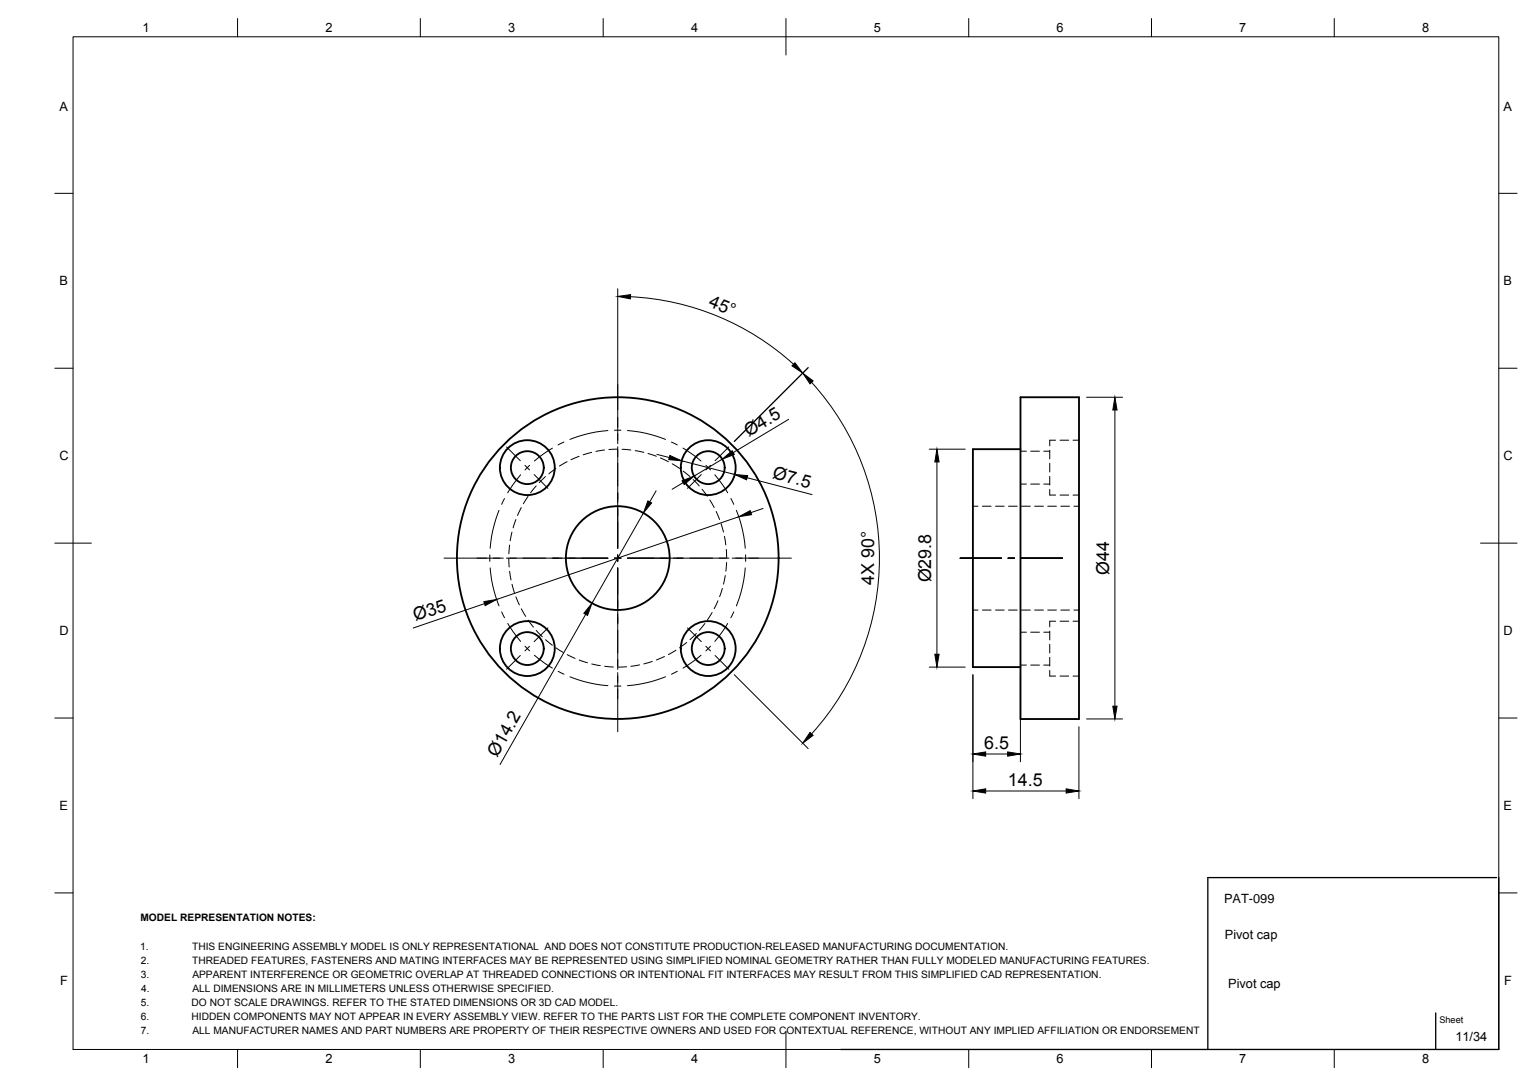
ISO-10303-21;
HEADER;
/* Generated by software containing ST-Developer
 * from STEP Tools, Inc. (www.steptools.com) 
 */

FILE_DESCRIPTION(
/* description */ ('PAT-099'),
/* implementation_level */ '2;1');

FILE_NAME(
/* name */ 'Pivot cap.step',
/* time_stamp */ '2026-10-29T17:25:42-07:00',
/* author */ (''),
/* organization */ (''),
/* preprocessor_version */ 'ST-DEVELOPER v20.2',
/* originating_system */ 'Autodesk Translation Framework v15.17.0.0',
/* authorisation */ '');

FILE_SCHEMA (('AUTOMOTIVE_DESIGN { 1 0 10303 214 3 1 1 }'));
ENDSEC;

DATA;
#10=MECHANICAL_DESIGN_GEOMETRIC_PRESENTATION_REPRESENTATION('',(#343),#11035);
#293=SHAPE_REPRESENTATION_RELATIONSHIP('SRR','None',#11161,#318);
#318=ADVANCED_BREP_SHAPE_REPRESENTATION('',(#376),#11011);
#343=STYLED_ITEM('',(#11372),#376);
#376=MANIFOLD_SOLID_BREP('Body1',#4711);
#463=FACE_BOUND('',#1091,.T.);
#464=FACE_BOUND('',#1094,.T.);
#465=FACE_BOUND('',#1097,.T.);
#466=FACE_BOUND('',#1100,.T.);
#467=FACE_BOUND('',#1107,.T.);
#468=FACE_BOUND('',#1111,.T.);
#469=FACE_BOUND('',#1112,.T.);
#470=FACE_BOUND('',#1113,.T.);
#471=FACE_BOUND('',#1114,.T.);
#472=FACE_BOUND('',#1115,.T.);
#473=FACE_BOUND('',#1117,.T.);
#474=FACE_BOUND('',#1118,.T.);
#475=FACE_BOUND('',#1119,.T.);
#476=FACE_BOUND('',#1120,.T.);
#477=FACE_BOUND('',#1121,.T.);
#555=PLANE('',#5222);
#556=PLANE('',#5227);
#557=PLANE('',#5232);
#558=PLANE('',#5237);
#559=PLANE('',#5250);
#560=PLANE('',#5257);
#561=PLANE('',#5258);
#746=FACE_OUTER_BOUND('',#1089,.T.);
#747=FACE_OUTER_BOUND('',#1090,.T.);
#748=FACE_OUTER_BOUND('',#1092,.T.);
#749=FACE_OUTER_BOUND('',#1093,.T.);
#750=FACE_OUTER_BOUND('',#1095,.T.);
#751=FACE_OUTER_BOUND('',#1096,.T.);
#752=FACE_OUTER_BOUND('',#1098,.T.);
#753=FACE_OUTER_BOUND('',#1099,.T.);
#754=FACE_OUTER_BOUND('',#1101,.T.);
#755=FACE_OUTER_BOUND('',#1102,.T.);
#756=FACE_OUTER_BOUND('',#1103,.T.);
#757=FACE_OUTER_BOUND('',#1104,.T.);
#758=FACE_OUTER_BOUND('',#1105,.T.);
#759=FACE_OUTER_BOUND('',#1106,.T.);
#760=FACE_OUTER_BOUND('',#1108,.T.);
#761=FACE_OUTER_BOUND('',#1109,.T.);
#762=FACE_OUTER_BOUND('',#1110,.T.);
#763=FACE_OUTER_BOUND('',#1116,.T.);
#1089=EDGE_LOOP('',(#3557,#3558,#3559,#3560));
#1090=EDGE_LOOP('',(#3561));
#1091=EDGE_LOOP('',(#3562));
#1092=EDGE_LOOP('',(#3563,#3564,#3565,#3566));
#1093=EDGE_LOOP('',(#3567));
#1094=EDGE_LOOP('',(#3568));
#1095=EDGE_LOOP('',(#3569,#3570,#3571,#3572));
#1096=EDGE_LOOP('',(#3573));
#1097=EDGE_LOOP('',(#3574));
#1098=EDGE_LOOP('',(#3575,#3576,#3577,#3578));
#1099=EDGE_LOOP('',(#3579));
#1100=EDGE_LOOP('',(#3580));
#1101=EDGE_LOOP('',(#3581,#3582,#3583,#3584));
#1102=EDGE_LOOP('',(#3585,#3586,#3587,#3588));
#1103=EDGE_LOOP('',(#3589,#3590,#3591,#3592));
#1104=EDGE_LOOP('',(#3593,#3594,#3595,#3596));
#1105=EDGE_LOOP('',(#3597,#3598,#3599,#3600));
#1106=EDGE_LOOP('',(#3601));
#1107=EDGE_LOOP('',(#3602));
#1108=EDGE_LOOP('',(#3603,#3604,#3605,#3606));
#1109=EDGE_LOOP('',(#3607,#3608,#3609,#3610));
#1110=EDGE_LOOP('',(#3611));
#1111=EDGE_LOOP('',(#3612));
#1112=EDGE_LOOP('',(#3613));
#1113=EDGE_LOOP('',(#3614));
#1114=EDGE_LOOP('',(#3615));
#1115=EDGE_LOOP('',(#3616));
#1116=EDGE_LOOP('',(#3617));
#1117=EDGE_LOOP('',(#3618));
#1118=EDGE_LOOP('',(#3619));
#1119=EDGE_LOOP('',(#3620));
#1120=EDGE_LOOP('',(#3621));
#1121=EDGE_LOOP('',(#3622));
#1425=LINE('',#9675,#1677);
#1426=LINE('',#9684,#1678);
#1427=LINE('',#9693,#1679);
#1428=LINE('',#9702,#1680);
#1429=LINE('',#9710,#1681);
#1430=LINE('',#9714,#1682);
#1431=LINE('',#9718,#1683);
#1432=LINE('',#9722,#1684);
#1433=LINE('',#9727,#1685);
#1434=LINE('',#9735,#1686);
#1435=LINE('',#9740,#1687);
#1677=VECTOR('',#6160,0.375);
#1678=VECTOR('',#6171,0.375);
#1679=VECTOR('',#6182,0.375);
#1680=VECTOR('',#6193,0.375);
#1681=VECTOR('',#6204,0.225);
#1682=VECTOR('',#6209,0.225);
#1683=VECTOR('',#6214,0.225);
#1684=VECTOR('',#6219,0.225);
#1685=VECTOR('',#6224,1.49);
#1686=VECTOR('',#6235,0.71);
#1687=VECTOR('',#6240,2.2);
#1955=CIRCLE('',#5220,0.375);
#1956=CIRCLE('',#5221,0.375);
#1957=CIRCLE('',#5223,0.225);
#1958=CIRCLE('',#5225,0.375);
#1959=CIRCLE('',#5226,0.375);
#1960=CIRCLE('',#5228,0.225);
#1961=CIRCLE('',#5230,0.375);
#1962=CIRCLE('',#5231,0.375);
#1963=CIRCLE('',#5233,0.225);
#1964=CIRCLE('',#5235,0.375);
#1965=CIRCLE('',#5236,0.375);
#1966=CIRCLE('',#5238,0.225);
#1967=CIRCLE('',#5240,0.225);
#1968=CIRCLE('',#5242,0.225);
#1969=CIRCLE('',#5244,0.225);
#1970=CIRCLE('',#5246,0.225);
#1971=CIRCLE('',#5248,1.49);
#1972=CIRCLE('',#5249,1.49);
#1973=CIRCLE('',#5251,0.71);
#1974=CIRCLE('',#5253,0.71);
#1975=CIRCLE('',#5255,2.2);
#1976=CIRCLE('',#5256,2.2);
#2284=VERTEX_POINT('',#9672);
#2285=VERTEX_POINT('',#9674);
#2286=VERTEX_POINT('',#9678);
#2287=VERTEX_POINT('',#9681);
#2288=VERTEX_POINT('',#9683);
#2289=VERTEX_POINT('',#9687);
#2290=VERTEX_POINT('',#9690);
#2291=VERTEX_POINT('',#9692);
#2292=VERTEX_POINT('',#9696);
#2293=VERTEX_POINT('',#9699);
#2294=VERTEX_POINT('',#9701);
#2295=VERTEX_POINT('',#9705);
#2296=VERTEX_POINT('',#9708);
#2297=VERTEX_POINT('',#9712);
#2298=VERTEX_POINT('',#9716);
#2299=VERTEX_POINT('',#9720);
#2300=VERTEX_POINT('',#9724);
#2301=VERTEX_POINT('',#9726);
#2302=VERTEX_POINT('',#9730);
#2303=VERTEX_POINT('',#9733);
#2304=VERTEX_POINT('',#9737);
#2305=VERTEX_POINT('',#9739);
#2755=EDGE_CURVE('',#2284,#2284,#1955,.T.);
#2756=EDGE_CURVE('',#2284,#2285,#1425,.T.);
#2757=EDGE_CURVE('',#2285,#2285,#1956,.T.);
#2758=EDGE_CURVE('',#2286,#2286,#1957,.T.);
#2759=EDGE_CURVE('',#2287,#2287,#1958,.T.);
#2760=EDGE_CURVE('',#2287,#2288,#1426,.T.);
#2761=EDGE_CURVE('',#2288,#2288,#1959,.T.);
#2762=EDGE_CURVE('',#2289,#2289,#1960,.T.);
#2763=EDGE_CURVE('',#2290,#2290,#1961,.T.);
#2764=EDGE_CURVE('',#2290,#2291,#1427,.T.);
#2765=EDGE_CURVE('',#2291,#2291,#1962,.T.);
#2766=EDGE_CURVE('',#2292,#2292,#1963,.T.);
#2767=EDGE_CURVE('',#2293,#2293,#1964,.T.);
#2768=EDGE_CURVE('',#2293,#2294,#1428,.T.);
#2769=EDGE_CURVE('',#2294,#2294,#1965,.T.);
#2770=EDGE_CURVE('',#2295,#2295,#1966,.T.);
#2771=EDGE_CURVE('',#2296,#2296,#1967,.T.);
#2772=EDGE_CURVE('',#2296,#2286,#1429,.T.);
#2773=EDGE_CURVE('',#2297,#2297,#1968,.T.);
#2774=EDGE_CURVE('',#2297,#2289,#1430,.T.);
#2775=EDGE_CURVE('',#2298,#2298,#1969,.T.);
#2776=EDGE_CURVE('',#2298,#2292,#1431,.T.);
#2777=EDGE_CURVE('',#2299,#2299,#1970,.T.);
#2778=EDGE_CURVE('',#2299,#2295,#1432,.T.);
#2779=EDGE_CURVE('',#2300,#2300,#1971,.T.);
#2780=EDGE_CURVE('',#2300,#2301,#1433,.T.);
#2781=EDGE_CURVE('',#2301,#2301,#1972,.T.);
#2782=EDGE_CURVE('',#2302,#2302,#1973,.T.);
#2783=EDGE_CURVE('',#2303,#2303,#1974,.T.);
#2784=EDGE_CURVE('',#2303,#2302,#1434,.T.);
#2785=EDGE_CURVE('',#2304,#2304,#1975,.T.);
#2786=EDGE_CURVE('',#2304,#2305,#1435,.T.);
#2787=EDGE_CURVE('',#2305,#2305,#1976,.T.);
#3557=ORIENTED_EDGE('',*,*,#2755,.F.);
#3558=ORIENTED_EDGE('',*,*,#2756,.T.);
#3559=ORIENTED_EDGE('',*,*,#2757,.F.);
#3560=ORIENTED_EDGE('',*,*,#2756,.F.);
#3561=ORIENTED_EDGE('',*,*,#2755,.T.);
#3562=ORIENTED_EDGE('',*,*,#2758,.F.);
#3563=ORIENTED_EDGE('',*,*,#2759,.F.);
#3564=ORIENTED_EDGE('',*,*,#2760,.T.);
#3565=ORIENTED_EDGE('',*,*,#2761,.F.);
#3566=ORIENTED_EDGE('',*,*,#2760,.F.);
#3567=ORIENTED_EDGE('',*,*,#2759,.T.);
#3568=ORIENTED_EDGE('',*,*,#2762,.F.);
#3569=ORIENTED_EDGE('',*,*,#2763,.F.);
#3570=ORIENTED_EDGE('',*,*,#2764,.T.);
#3571=ORIENTED_EDGE('',*,*,#2765,.F.);
#3572=ORIENTED_EDGE('',*,*,#2764,.F.);
#3573=ORIENTED_EDGE('',*,*,#2763,.T.);
#3574=ORIENTED_EDGE('',*,*,#2766,.F.);
#3575=ORIENTED_EDGE('',*,*,#2767,.F.);
#3576=ORIENTED_EDGE('',*,*,#2768,.T.);
#3577=ORIENTED_EDGE('',*,*,#2769,.F.);
#3578=ORIENTED_EDGE('',*,*,#2768,.F.);
#3579=ORIENTED_EDGE('',*,*,#2767,.T.);
#3580=ORIENTED_EDGE('',*,*,#2770,.F.);
#3581=ORIENTED_EDGE('',*,*,#2771,.F.);
#3582=ORIENTED_EDGE('',*,*,#2772,.T.);
#3583=ORIENTED_EDGE('',*,*,#2758,.T.);
#3584=ORIENTED_EDGE('',*,*,#2772,.F.);
#3585=ORIENTED_EDGE('',*,*,#2773,.F.);
#3586=ORIENTED_EDGE('',*,*,#2774,.T.);
#3587=ORIENTED_EDGE('',*,*,#2762,.T.);
#3588=ORIENTED_EDGE('',*,*,#2774,.F.);
#3589=ORIENTED_EDGE('',*,*,#2775,.F.);
#3590=ORIENTED_EDGE('',*,*,#2776,.T.);
#3591=ORIENTED_EDGE('',*,*,#2766,.T.);
#3592=ORIENTED_EDGE('',*,*,#2776,.F.);
#3593=ORIENTED_EDGE('',*,*,#2777,.F.);
#3594=ORIENTED_EDGE('',*,*,#2778,.T.);
#3595=ORIENTED_EDGE('',*,*,#2770,.T.);
#3596=ORIENTED_EDGE('',*,*,#2778,.F.);
#3597=ORIENTED_EDGE('',*,*,#2779,.F.);
#3598=ORIENTED_EDGE('',*,*,#2780,.T.);
#3599=ORIENTED_EDGE('',*,*,#2781,.T.);
#3600=ORIENTED_EDGE('',*,*,#2780,.F.);
#3601=ORIENTED_EDGE('',*,*,#2781,.F.);
#3602=ORIENTED_EDGE('',*,*,#2782,.F.);
#3603=ORIENTED_EDGE('',*,*,#2783,.F.);
#3604=ORIENTED_EDGE('',*,*,#2784,.T.);
#3605=ORIENTED_EDGE('',*,*,#2782,.T.);
#3606=ORIENTED_EDGE('',*,*,#2784,.F.);
#3607=ORIENTED_EDGE('',*,*,#2785,.F.);
#3608=ORIENTED_EDGE('',*,*,#2786,.T.);
#3609=ORIENTED_EDGE('',*,*,#2787,.T.);
#3610=ORIENTED_EDGE('',*,*,#2786,.F.);
#3611=ORIENTED_EDGE('',*,*,#2785,.T.);
#3612=ORIENTED_EDGE('',*,*,#2783,.T.);
#3613=ORIENTED_EDGE('',*,*,#2769,.T.);
#3614=ORIENTED_EDGE('',*,*,#2765,.T.);
#3615=ORIENTED_EDGE('',*,*,#2761,.T.);
#3616=ORIENTED_EDGE('',*,*,#2757,.T.);
#3617=ORIENTED_EDGE('',*,*,#2787,.F.);
#3618=ORIENTED_EDGE('',*,*,#2779,.T.);
#3619=ORIENTED_EDGE('',*,*,#2777,.T.);
#3620=ORIENTED_EDGE('',*,*,#2775,.T.);
#3621=ORIENTED_EDGE('',*,*,#2773,.T.);
#3622=ORIENTED_EDGE('',*,*,#2771,.T.);
#4363=CYLINDRICAL_SURFACE('',#5219,0.375);
#4364=CYLINDRICAL_SURFACE('',#5224,0.375);
#4365=CYLINDRICAL_SURFACE('',#5229,0.375);
#4366=CYLINDRICAL_SURFACE('',#5234,0.375);
#4367=CYLINDRICAL_SURFACE('',#5239,0.225);
#4368=CYLINDRICAL_SURFACE('',#5241,0.225);
#4369=CYLINDRICAL_SURFACE('',#5243,0.225);
#4370=CYLINDRICAL_SURFACE('',#5245,0.225);
#4371=CYLINDRICAL_SURFACE('',#5247,1.49);
#4372=CYLINDRICAL_SURFACE('',#5252,0.71);
#4373=CYLINDRICAL_SURFACE('',#5254,2.2);
#4511=ADVANCED_FACE('',(#746),#4363,.F.);
#4512=ADVANCED_FACE('',(#747,#463),#555,.T.);
#4513=ADVANCED_FACE('',(#748),#4364,.F.);
#4514=ADVANCED_FACE('',(#749,#464),#556,.T.);
#4515=ADVANCED_FACE('',(#750),#4365,.F.);
#4516=ADVANCED_FACE('',(#751,#465),#557,.T.);
#4517=ADVANCED_FACE('',(#752),#4366,.F.);
#4518=ADVANCED_FACE('',(#753,#466),#558,.T.);
#4519=ADVANCED_FACE('',(#754),#4367,.F.);
#4520=ADVANCED_FACE('',(#755),#4368,.F.);
#4521=ADVANCED_FACE('',(#756),#4369,.F.);
#4522=ADVANCED_FACE('',(#757),#4370,.F.);
#4523=ADVANCED_FACE('',(#758),#4371,.T.);
#4524=ADVANCED_FACE('',(#759,#467),#559,.F.);
#4525=ADVANCED_FACE('',(#760),#4372,.F.);
#4526=ADVANCED_FACE('',(#761),#4373,.T.);
#4527=ADVANCED_FACE('',(#762,#468,#469,#470,#471,#472),#560,.T.);
#4528=ADVANCED_FACE('',(#763,#473,#474,#475,#476,#477),#561,.F.);
#4711=CLOSED_SHELL('',(#4511,#4512,#4513,#4514,#4515,#4516,#4517,#4518,
#4519,#4520,#4521,#4522,#4523,#4524,#4525,#4526,#4527,#4528));
#5218=AXIS2_PLACEMENT_3D('',#9670,#6154,#6155);
#5219=AXIS2_PLACEMENT_3D('',#9671,#6156,#6157);
#5220=AXIS2_PLACEMENT_3D('',#9673,#6158,#6159);
#5221=AXIS2_PLACEMENT_3D('',#9676,#6161,#6162);
#5222=AXIS2_PLACEMENT_3D('',#9677,#6163,#6164);
#5223=AXIS2_PLACEMENT_3D('',#9679,#6165,#6166);
#5224=AXIS2_PLACEMENT_3D('',#9680,#6167,#6168);
#5225=AXIS2_PLACEMENT_3D('',#9682,#6169,#6170);
#5226=AXIS2_PLACEMENT_3D('',#9685,#6172,#6173);
#5227=AXIS2_PLACEMENT_3D('',#9686,#6174,#6175);
#5228=AXIS2_PLACEMENT_3D('',#9688,#6176,#6177);
#5229=AXIS2_PLACEMENT_3D('',#9689,#6178,#6179);
#5230=AXIS2_PLACEMENT_3D('',#9691,#6180,#6181);
#5231=AXIS2_PLACEMENT_3D('',#9694,#6183,#6184);
#5232=AXIS2_PLACEMENT_3D('',#9695,#6185,#6186);
#5233=AXIS2_PLACEMENT_3D('',#9697,#6187,#6188);
#5234=AXIS2_PLACEMENT_3D('',#9698,#6189,#6190);
#5235=AXIS2_PLACEMENT_3D('',#9700,#6191,#6192);
#5236=AXIS2_PLACEMENT_3D('',#9703,#6194,#6195);
#5237=AXIS2_PLACEMENT_3D('',#9704,#6196,#6197);
#5238=AXIS2_PLACEMENT_3D('',#9706,#6198,#6199);
#5239=AXIS2_PLACEMENT_3D('',#9707,#6200,#6201);
#5240=AXIS2_PLACEMENT_3D('',#9709,#6202,#6203);
#5241=AXIS2_PLACEMENT_3D('',#9711,#6205,#6206);
#5242=AXIS2_PLACEMENT_3D('',#9713,#6207,#6208);
#5243=AXIS2_PLACEMENT_3D('',#9715,#6210,#6211);
#5244=AXIS2_PLACEMENT_3D('',#9717,#6212,#6213);
#5245=AXIS2_PLACEMENT_3D('',#9719,#6215,#6216);
#5246=AXIS2_PLACEMENT_3D('',#9721,#6217,#6218);
#5247=AXIS2_PLACEMENT_3D('',#9723,#6220,#6221);
#5248=AXIS2_PLACEMENT_3D('',#9725,#6222,#6223);
#5249=AXIS2_PLACEMENT_3D('',#9728,#6225,#6226);
#5250=AXIS2_PLACEMENT_3D('',#9729,#6227,#6228);
#5251=AXIS2_PLACEMENT_3D('',#9731,#6229,#6230);
#5252=AXIS2_PLACEMENT_3D('',#9732,#6231,#6232);
#5253=AXIS2_PLACEMENT_3D('',#9734,#6233,#6234);
#5254=AXIS2_PLACEMENT_3D('',#9736,#6236,#6237);
#5255=AXIS2_PLACEMENT_3D('',#9738,#6238,#6239);
#5256=AXIS2_PLACEMENT_3D('',#9741,#6241,#6242);
#5257=AXIS2_PLACEMENT_3D('',#9742,#6243,#6244);
#5258=AXIS2_PLACEMENT_3D('',#9743,#6245,#6246);
#6154=DIRECTION('axis',(0.,0.,1.));
#6155=DIRECTION('refdir',(1.,0.,0.));
#6156=DIRECTION('center_axis',(0.,0.,1.));
#6157=DIRECTION('ref_axis',(1.,0.,0.));
#6158=DIRECTION('center_axis',(0.,0.,1.));
#6159=DIRECTION('ref_axis',(1.,0.,0.));
#6160=DIRECTION('',(0.,0.,1.));
#6161=DIRECTION('center_axis',(0.,0.,-1.));
#6162=DIRECTION('ref_axis',(1.,0.,0.));
#6163=DIRECTION('center_axis',(0.,0.,1.));
#6164=DIRECTION('ref_axis',(1.,0.,0.));
#6165=DIRECTION('center_axis',(0.,0.,1.));
#6166=DIRECTION('ref_axis',(1.,0.,0.));
#6167=DIRECTION('center_axis',(0.,0.,1.));
#6168=DIRECTION('ref_axis',(1.,0.,0.));
#6169=DIRECTION('center_axis',(0.,0.,1.));
#6170=DIRECTION('ref_axis',(1.,0.,0.));
#6171=DIRECTION('',(0.,0.,1.));
#6172=DIRECTION('center_axis',(0.,0.,-1.));
#6173=DIRECTION('ref_axis',(1.,0.,0.));
#6174=DIRECTION('center_axis',(0.,0.,1.));
#6175=DIRECTION('ref_axis',(1.,0.,0.));
#6176=DIRECTION('center_axis',(0.,0.,1.));
#6177=DIRECTION('ref_axis',(1.,0.,0.));
#6178=DIRECTION('center_axis',(0.,0.,1.));
#6179=DIRECTION('ref_axis',(1.,0.,0.));
#6180=DIRECTION('center_axis',(0.,0.,1.));
#6181=DIRECTION('ref_axis',(1.,0.,0.));
#6182=DIRECTION('',(0.,0.,1.));
#6183=DIRECTION('center_axis',(0.,0.,-1.));
#6184=DIRECTION('ref_axis',(1.,0.,0.));
#6185=DIRECTION('center_axis',(0.,0.,1.));
#6186=DIRECTION('ref_axis',(1.,0.,0.));
#6187=DIRECTION('center_axis',(0.,0.,1.));
#6188=DIRECTION('ref_axis',(1.,0.,0.));
#6189=DIRECTION('center_axis',(0.,0.,1.));
#6190=DIRECTION('ref_axis',(1.,0.,0.));
#6191=DIRECTION('center_axis',(0.,0.,1.));
#6192=DIRECTION('ref_axis',(1.,0.,0.));
#6193=DIRECTION('',(0.,0.,1.));
#6194=DIRECTION('center_axis',(0.,0.,-1.));
#6195=DIRECTION('ref_axis',(1.,0.,0.));
#6196=DIRECTION('center_axis',(0.,0.,1.));
#6197=DIRECTION('ref_axis',(1.,0.,0.));
#6198=DIRECTION('center_axis',(0.,0.,1.));
#6199=DIRECTION('ref_axis',(1.,0.,0.));
#6200=DIRECTION('center_axis',(0.,0.,1.));
#6201=DIRECTION('ref_axis',(1.,0.,0.));
#6202=DIRECTION('center_axis',(0.,0.,1.));
#6203=DIRECTION('ref_axis',(1.,0.,0.));
#6204=DIRECTION('',(0.,0.,1.));
#6205=DIRECTION('center_axis',(0.,0.,1.));
#6206=DIRECTION('ref_axis',(1.,0.,0.));
#6207=DIRECTION('center_axis',(0.,0.,1.));
#6208=DIRECTION('ref_axis',(1.,0.,0.));
#6209=DIRECTION('',(0.,0.,1.));
#6210=DIRECTION('center_axis',(0.,0.,1.));
#6211=DIRECTION('ref_axis',(1.,0.,0.));
#6212=DIRECTION('center_axis',(0.,0.,1.));
#6213=DIRECTION('ref_axis',(1.,0.,0.));
#6214=DIRECTION('',(0.,0.,1.));
#6215=DIRECTION('center_axis',(0.,0.,1.));
#6216=DIRECTION('ref_axis',(1.,0.,0.));
#6217=DIRECTION('center_axis',(0.,0.,1.));
#6218=DIRECTION('ref_axis',(1.,0.,0.));
#6219=DIRECTION('',(0.,0.,1.));
#6220=DIRECTION('center_axis',(0.,0.,1.));
#6221=DIRECTION('ref_axis',(1.,0.,0.));
#6222=DIRECTION('center_axis',(0.,0.,1.));
#6223=DIRECTION('ref_axis',(1.,0.,0.));
#6224=DIRECTION('',(0.,0.,-1.));
#6225=DIRECTION('center_axis',(0.,0.,1.));
#6226=DIRECTION('ref_axis',(1.,0.,0.));
#6227=DIRECTION('center_axis',(0.,0.,1.));
#6228=DIRECTION('ref_axis',(1.,0.,0.));
#6229=DIRECTION('center_axis',(0.,0.,-1.));
#6230=DIRECTION('ref_axis',(1.,0.,0.));
#6231=DIRECTION('center_axis',(0.,0.,1.));
#6232=DIRECTION('ref_axis',(1.,0.,0.));
#6233=DIRECTION('center_axis',(0.,0.,-1.));
#6234=DIRECTION('ref_axis',(1.,0.,0.));
#6235=DIRECTION('',(0.,0.,-1.));
#6236=DIRECTION('center_axis',(0.,0.,1.));
#6237=DIRECTION('ref_axis',(1.,0.,0.));
#6238=DIRECTION('center_axis',(0.,0.,1.));
#6239=DIRECTION('ref_axis',(1.,0.,0.));
#6240=DIRECTION('',(0.,0.,-1.));
#6241=DIRECTION('center_axis',(0.,0.,1.));
#6242=DIRECTION('ref_axis',(1.,0.,0.));
#6243=DIRECTION('center_axis',(0.,0.,1.));
#6244=DIRECTION('ref_axis',(1.,0.,0.));
#6245=DIRECTION('center_axis',(0.,0.,1.));
#6246=DIRECTION('ref_axis',(1.,0.,0.));
#9670=CARTESIAN_POINT('',(0.,0.,0.));
#9671=CARTESIAN_POINT('Origin',(-1.23743686707646,-1.23743686707646,4.));
#9672=CARTESIAN_POINT('',(-1.61243686707646,-1.23743686707646,4.));
#9673=CARTESIAN_POINT('Origin',(-1.23743686707646,-1.23743686707646,4.));
#9674=CARTESIAN_POINT('',(-1.61243686707646,-1.23743686707646,4.4));
#9675=CARTESIAN_POINT('',(-1.61243686707646,-1.23743686707646,4.));
#9676=CARTESIAN_POINT('Origin',(-1.23743686707646,-1.23743686707646,4.4));
#9677=CARTESIAN_POINT('Origin',(-1.23743686707646,-1.23743686707646,4.));
#9678=CARTESIAN_POINT('',(-1.46243686707646,-1.23743686707646,4.));
#9679=CARTESIAN_POINT('Origin',(-1.23743686707646,-1.23743686707646,4.));
#9680=CARTESIAN_POINT('Origin',(-1.23743686707646,1.23743686707646,4.));
#9681=CARTESIAN_POINT('',(-1.61243686707646,1.23743686707646,4.));
#9682=CARTESIAN_POINT('Origin',(-1.23743686707646,1.23743686707646,4.));
#9683=CARTESIAN_POINT('',(-1.61243686707646,1.23743686707646,4.4));
#9684=CARTESIAN_POINT('',(-1.61243686707646,1.23743686707646,4.));
#9685=CARTESIAN_POINT('Origin',(-1.23743686707646,1.23743686707646,4.4));
#9686=CARTESIAN_POINT('Origin',(-1.23743686707646,1.23743686707646,4.));
#9687=CARTESIAN_POINT('',(-1.46243686707646,1.23743686707646,4.));
#9688=CARTESIAN_POINT('Origin',(-1.23743686707646,1.23743686707646,4.));
#9689=CARTESIAN_POINT('Origin',(1.23743686707646,1.23743686707646,4.));
#9690=CARTESIAN_POINT('',(0.862436867076458,1.23743686707646,4.));
#9691=CARTESIAN_POINT('Origin',(1.23743686707646,1.23743686707646,4.));
#9692=CARTESIAN_POINT('',(0.862436867076458,1.23743686707646,4.4));
#9693=CARTESIAN_POINT('',(0.862436867076458,1.23743686707646,4.));
#9694=CARTESIAN_POINT('Origin',(1.23743686707646,1.23743686707646,4.4));
#9695=CARTESIAN_POINT('Origin',(1.23743686707646,1.23743686707646,4.));
#9696=CARTESIAN_POINT('',(1.01243686707646,1.23743686707646,4.));
#9697=CARTESIAN_POINT('Origin',(1.23743686707646,1.23743686707646,4.));
#9698=CARTESIAN_POINT('Origin',(1.23743686707646,-1.23743686707646,4.));
#9699=CARTESIAN_POINT('',(0.862436867076458,-1.23743686707646,4.));
#9700=CARTESIAN_POINT('Origin',(1.23743686707646,-1.23743686707646,4.));
#9701=CARTESIAN_POINT('',(0.862436867076458,-1.23743686707646,4.4));
#9702=CARTESIAN_POINT('',(0.862436867076458,-1.23743686707646,4.));
#9703=CARTESIAN_POINT('Origin',(1.23743686707646,-1.23743686707646,4.4));
#9704=CARTESIAN_POINT('Origin',(1.23743686707646,-1.23743686707646,4.));
#9705=CARTESIAN_POINT('',(1.01243686707646,-1.23743686707646,4.));
#9706=CARTESIAN_POINT('Origin',(1.23743686707646,-1.23743686707646,4.));
#9707=CARTESIAN_POINT('Origin',(-1.23743686707646,-1.23743686707646,3.5));
#9708=CARTESIAN_POINT('',(-1.46243686707646,-1.23743686707646,3.6));
#9709=CARTESIAN_POINT('Origin',(-1.23743686707646,-1.23743686707646,3.6));
#9710=CARTESIAN_POINT('',(-1.46243686707646,-1.23743686707646,3.5));
#9711=CARTESIAN_POINT('Origin',(-1.23743686707646,1.23743686707646,3.5));
#9712=CARTESIAN_POINT('',(-1.46243686707646,1.23743686707646,3.6));
#9713=CARTESIAN_POINT('Origin',(-1.23743686707646,1.23743686707646,3.6));
#9714=CARTESIAN_POINT('',(-1.46243686707646,1.23743686707646,3.5));
#9715=CARTESIAN_POINT('Origin',(1.23743686707646,1.23743686707646,3.5));
#9716=CARTESIAN_POINT('',(1.01243686707646,1.23743686707646,3.6));
#9717=CARTESIAN_POINT('Origin',(1.23743686707646,1.23743686707646,3.6));
#9718=CARTESIAN_POINT('',(1.01243686707646,1.23743686707646,3.5));
#9719=CARTESIAN_POINT('Origin',(1.23743686707646,-1.23743686707646,3.5));
#9720=CARTESIAN_POINT('',(1.01243686707646,-1.23743686707646,3.6));
#9721=CARTESIAN_POINT('Origin',(1.23743686707646,-1.23743686707646,3.6));
#9722=CARTESIAN_POINT('',(1.01243686707646,-1.23743686707646,3.5));
#9723=CARTESIAN_POINT('Origin',(0.,0.,2.95));
#9724=CARTESIAN_POINT('',(-1.49,-1.82472373072956E-16,3.6));
#9725=CARTESIAN_POINT('Origin',(0.,0.,3.6));
#9726=CARTESIAN_POINT('',(-1.49,-1.82472373072956E-16,2.95));
#9727=CARTESIAN_POINT('',(-1.49,-1.82472373072956E-16,2.95));
#9728=CARTESIAN_POINT('Origin',(0.,0.,2.95));
#9729=CARTESIAN_POINT('Origin',(0.,0.,2.95));
#9730=CARTESIAN_POINT('',(-0.71,-8.69499227394621E-17,2.95));
#9731=CARTESIAN_POINT('Origin',(0.,0.,2.95));
#9732=CARTESIAN_POINT('Origin',(0.,0.,3.6));
#9733=CARTESIAN_POINT('',(-0.71,-8.69499227394621E-17,4.4));
#9734=CARTESIAN_POINT('Origin',(0.,0.,4.4));
#9735=CARTESIAN_POINT('',(-0.71,-8.69499227394621E-17,3.6));
#9736=CARTESIAN_POINT('Origin',(0.,0.,3.6));
#9737=CARTESIAN_POINT('',(-2.2,-2.69422295812418E-16,4.4));
#9738=CARTESIAN_POINT('Origin',(0.,0.,4.4));
#9739=CARTESIAN_POINT('',(-2.2,-2.69422295812418E-16,3.6));
#9740=CARTESIAN_POINT('',(-2.2,-2.69422295812418E-16,3.6));
#9741=CARTESIAN_POINT('Origin',(0.,0.,3.6));
#9742=CARTESIAN_POINT('Origin',(0.,0.,4.4));
#9743=CARTESIAN_POINT('Origin',(0.,0.,3.6));
#10978=UNCERTAINTY_MEASURE_WITH_UNIT(LENGTH_MEASURE(0.001),#11036,
'DISTANCE_ACCURACY_VALUE',
'Maximum model space distance between geometric entities at asserted c
onnectivities');
#11002=UNCERTAINTY_MEASURE_WITH_UNIT(LENGTH_MEASURE(0.001),#11036,
'DISTANCE_ACCURACY_VALUE',
'Maximum model space distance between geometric entities at asserted c
onnectivities');
#11011=(
GEOMETRIC_REPRESENTATION_CONTEXT(3)
GLOBAL_UNCERTAINTY_ASSIGNED_CONTEXT((#10978))
GLOBAL_UNIT_ASSIGNED_CONTEXT((#11036,#11038,#11039))
REPRESENTATION_CONTEXT('','3D')
);
#11035=(
GEOMETRIC_REPRESENTATION_CONTEXT(3)
GLOBAL_UNCERTAINTY_ASSIGNED_CONTEXT((#11002))
GLOBAL_UNIT_ASSIGNED_CONTEXT((#11036,#11038,#11039))
REPRESENTATION_CONTEXT('','3D')
);
#11036=(
LENGTH_UNIT()
NAMED_UNIT(*)
SI_UNIT(.CENTI.,.METRE.)
);
#11038=(
NAMED_UNIT(*)
PLANE_ANGLE_UNIT()
SI_UNIT($,.RADIAN.)
);
#11039=(
NAMED_UNIT(*)
SI_UNIT($,.STERADIAN.)
SOLID_ANGLE_UNIT()
);
#11048=SHAPE_DEFINITION_REPRESENTATION(#11080,#11161);
#11080=PRODUCT_DEFINITION_SHAPE('',$,#11194);
#11161=SHAPE_REPRESENTATION('',(#5218),#11011);
#11185=PRODUCT_DEFINITION_CONTEXT('part definition',#11283,'design');
#11194=PRODUCT_DEFINITION('Pivot cap','Pivot cap',#11226,#11185);
#11226=PRODUCT_DEFINITION_FORMATION('',$,#11293);
#11283=APPLICATION_CONTEXT(
'Core Data for Automotive Mechanical Design Process');
#11284=PRODUCT_CONTEXT('part definition',#11283,'mechanical');
#11293=PRODUCT('Pivot cap','Pivot cap','Pivot cap',(#11284));
#11366=COLOUR_RGB('Light Blue',0.38,0.62,0.78);
#11367=FILL_AREA_STYLE_COLOUR('',#11366);
#11368=FILL_AREA_STYLE('',(#11367));
#11369=SURFACE_STYLE_FILL_AREA(#11368);
#11370=SURFACE_SIDE_STYLE('',(#11369));
#11371=SURFACE_STYLE_USAGE(.BOTH.,#11370);
#11372=PRESENTATION_STYLE_ASSIGNMENT((#11371));
ENDSEC;
END-ISO-10303-21;
